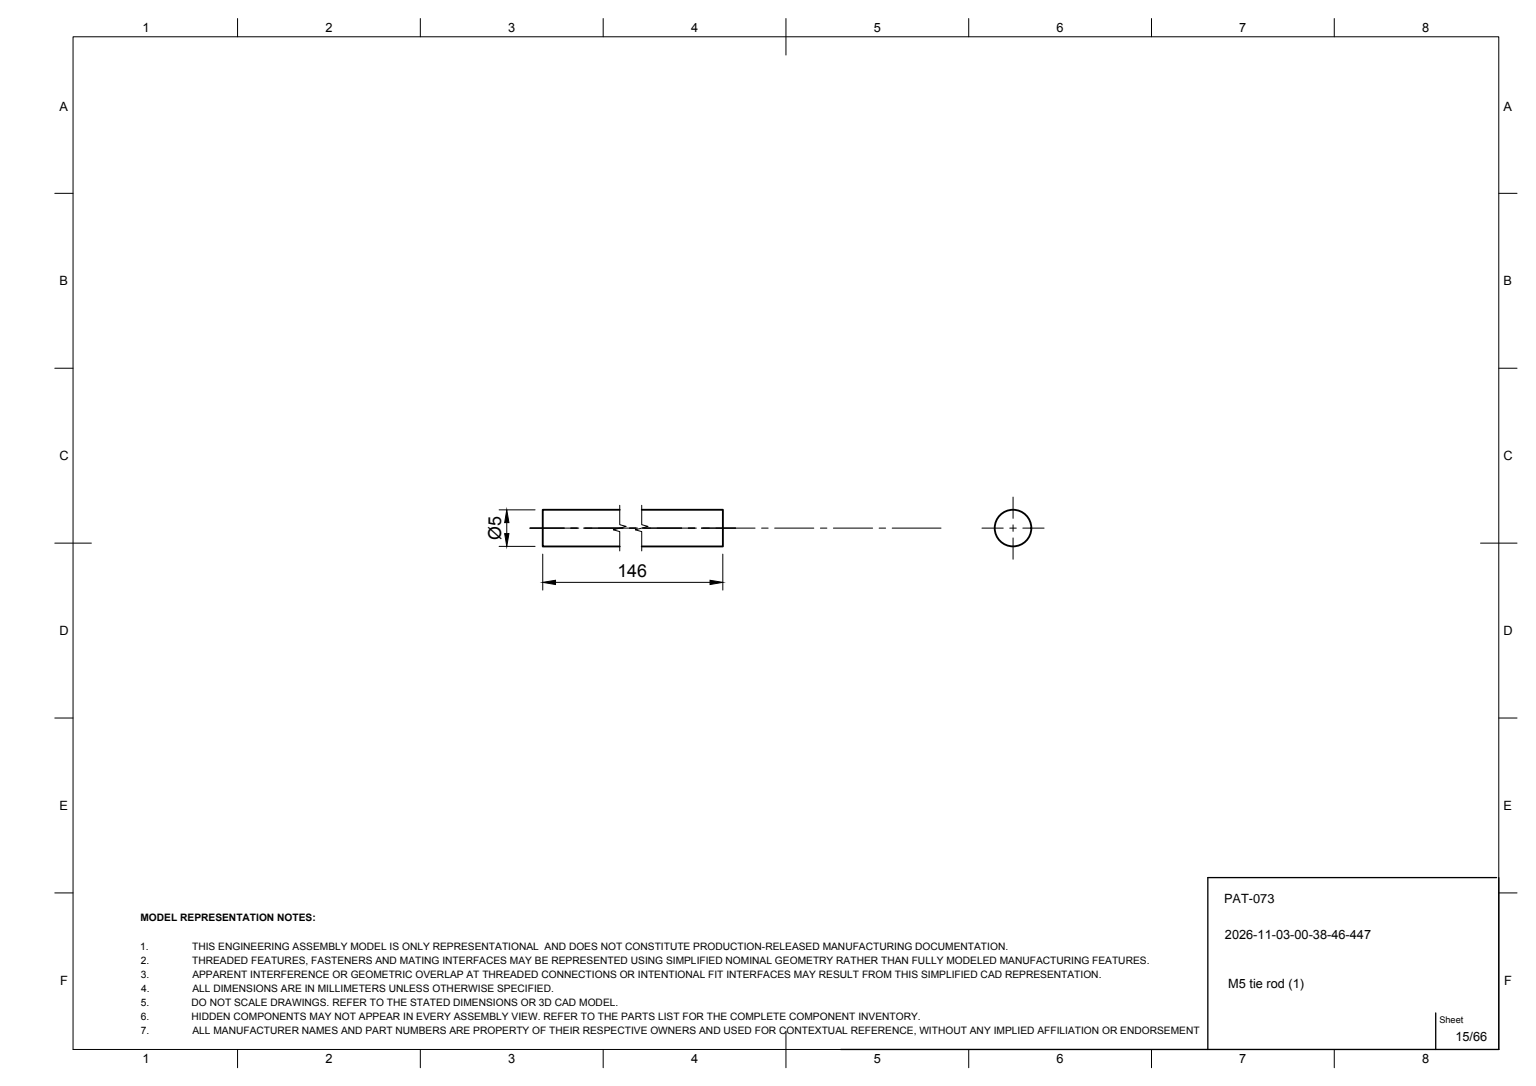
ISO-10303-21;
HEADER;
/* Generated by software containing ST-Developer
 * from STEP Tools, Inc. (www.steptools.com) 
 */

FILE_DESCRIPTION(
/* description */ ('Manual piston pump'),
/* implementation_level */ '2;1');

FILE_NAME(
/* name */ 'M5 tie rod (1).step',
/* time_stamp */ '2026-11-02T16:54:23-08:00',
/* author */ (''),
/* organization */ (''),
/* preprocessor_version */ 'ST-DEVELOPER v20.2',
/* originating_system */ 'Autodesk Translation Framework v15.17.0.0',
/* authorisation */ '');

FILE_SCHEMA (('AUTOMOTIVE_DESIGN { 1 0 10303 214 3 1 1 }'));
ENDSEC;

DATA;
#10=MECHANICAL_DESIGN_GEOMETRIC_PRESENTATION_REPRESENTATION('',(#698),#19043);
#572=SHAPE_REPRESENTATION_RELATIONSHIP('SRR','None',#19318,#635);
#635=ADVANCED_BREP_SHAPE_REPRESENTATION('',(#770),#18985);
#698=STYLED_ITEM('',(#19661),#770);
#770=MANIFOLD_SOLID_BREP('Body1',#9482);
#1139=CYLINDRICAL_SURFACE('',#10460,0.25);
#1396=FACE_OUTER_BOUND('',#2028,.T.);
#1397=FACE_OUTER_BOUND('',#2029,.T.);
#1398=FACE_OUTER_BOUND('',#2030,.T.);
#2028=EDGE_LOOP('',(#6717,#6718,#6719,#6720));
#2029=EDGE_LOOP('',(#6721));
#2030=EDGE_LOOP('',(#6722));
#2763=CIRCLE('',#10461,0.25);
#2764=CIRCLE('',#10462,0.25);
#3266=LINE('',#15144,#3870);
#3870=VECTOR('',#12052,0.25);
#4502=VERTEX_POINT('',#15141);
#4503=VERTEX_POINT('',#15143);
#5345=EDGE_CURVE('',#4502,#4502,#2763,.T.);
#5346=EDGE_CURVE('',#4502,#4503,#3266,.T.);
#5347=EDGE_CURVE('',#4503,#4503,#2764,.T.);
#6717=ORIENTED_EDGE('',*,*,#5345,.F.);
#6718=ORIENTED_EDGE('',*,*,#5346,.T.);
#6719=ORIENTED_EDGE('',*,*,#5347,.T.);
#6720=ORIENTED_EDGE('',*,*,#5346,.F.);
#6721=ORIENTED_EDGE('',*,*,#5345,.T.);
#6722=ORIENTED_EDGE('',*,*,#5347,.F.);
#8628=PLANE('',#10463);
#8629=PLANE('',#10464);
#9001=ADVANCED_FACE('',(#1396),#1139,.T.);
#9002=ADVANCED_FACE('',(#1397),#8628,.T.);
#9003=ADVANCED_FACE('',(#1398),#8629,.F.);
#9482=CLOSED_SHELL('',(#9001,#9002,#9003));
#10459=AXIS2_PLACEMENT_3D('',#15139,#12046,#12047);
#10460=AXIS2_PLACEMENT_3D('',#15140,#12048,#12049);
#10461=AXIS2_PLACEMENT_3D('',#15142,#12050,#12051);
#10462=AXIS2_PLACEMENT_3D('',#15145,#12053,#12054);
#10463=AXIS2_PLACEMENT_3D('',#15146,#12055,#12056);
#10464=AXIS2_PLACEMENT_3D('',#15147,#12057,#12058);
#12046=DIRECTION('axis',(0.,0.,1.));
#12047=DIRECTION('refdir',(1.,0.,0.));
#12048=DIRECTION('center_axis',(0.,1.,0.));
#12049=DIRECTION('ref_axis',(1.,0.,0.));
#12050=DIRECTION('center_axis',(0.,1.,0.));
#12051=DIRECTION('ref_axis',(1.,0.,0.));
#12052=DIRECTION('',(0.,-1.,0.));
#12053=DIRECTION('center_axis',(0.,1.,0.));
#12054=DIRECTION('ref_axis',(1.,0.,0.));
#12055=DIRECTION('center_axis',(0.,1.,0.));
#12056=DIRECTION('ref_axis',(1.,0.,0.));
#12057=DIRECTION('center_axis',(0.,1.,0.));
#12058=DIRECTION('ref_axis',(1.,0.,0.));
#15139=CARTESIAN_POINT('',(0.,0.,0.));
#15140=CARTESIAN_POINT('Origin',(-2.,-1.,6.5));
#15141=CARTESIAN_POINT('',(-2.25,13.6,6.5));
#15142=CARTESIAN_POINT('Origin',(-2.,13.6,6.5));
#15143=CARTESIAN_POINT('',(-2.25,-1.,6.5));
#15144=CARTESIAN_POINT('',(-2.25,-1.,6.5));
#15145=CARTESIAN_POINT('Origin',(-2.,-1.,6.5));
#15146=CARTESIAN_POINT('Origin',(-2.,13.6,6.5));
#15147=CARTESIAN_POINT('Origin',(-2.,-1.,6.5));
#18914=UNCERTAINTY_MEASURE_WITH_UNIT(LENGTH_MEASURE(0.001),#19044,
'DISTANCE_ACCURACY_VALUE',
'Maximum model space distance between geometric entities at asserted c
onnectivities');
#18972=UNCERTAINTY_MEASURE_WITH_UNIT(LENGTH_MEASURE(0.001),#19044,
'DISTANCE_ACCURACY_VALUE',
'Maximum model space distance between geometric entities at asserted c
onnectivities');
#18985=(
GEOMETRIC_REPRESENTATION_CONTEXT(3)
GLOBAL_UNCERTAINTY_ASSIGNED_CONTEXT((#18914))
GLOBAL_UNIT_ASSIGNED_CONTEXT((#19044,#19046,#19047))
REPRESENTATION_CONTEXT('','3D')
);
#19043=(
GEOMETRIC_REPRESENTATION_CONTEXT(3)
GLOBAL_UNCERTAINTY_ASSIGNED_CONTEXT((#18972))
GLOBAL_UNIT_ASSIGNED_CONTEXT((#19044,#19046,#19047))
REPRESENTATION_CONTEXT('','3D')
);
#19044=(
LENGTH_UNIT()
NAMED_UNIT(*)
SI_UNIT(.CENTI.,.METRE.)
);
#19046=(
NAMED_UNIT(*)
PLANE_ANGLE_UNIT()
SI_UNIT($,.RADIAN.)
);
#19047=(
NAMED_UNIT(*)
SI_UNIT($,.STERADIAN.)
SOLID_ANGLE_UNIT()
);
#19060=SHAPE_DEFINITION_REPRESENTATION(#19130,#19318);
#19130=PRODUCT_DEFINITION_SHAPE('',$,#19389);
#19318=SHAPE_REPRESENTATION('',(#10459),#18985);
#19376=PRODUCT_DEFINITION_CONTEXT('part definition',#19588,'design');
#19389=PRODUCT_DEFINITION('2026-11-03-00-38-46-447','M5 tie rod (1)',#19459,
#19376);
#19459=PRODUCT_DEFINITION_FORMATION('',$,#19602);
#19588=APPLICATION_CONTEXT(
'Core Data for Automotive Mechanical Design Process');
#19589=PRODUCT_CONTEXT('part definition',#19588,'mechanical');
#19602=PRODUCT('2026-11-03-00-38-46-447','M5 tie rod (1)','M5 tie rod',
(#19589));
#19661=PRESENTATION_STYLE_ASSIGNMENT((#19667));
#19667=SURFACE_STYLE_USAGE(.BOTH.,#19673);
#19673=SURFACE_SIDE_STYLE('',(#19679));
#19679=SURFACE_STYLE_FILL_AREA(#19685);
#19685=FILL_AREA_STYLE('CAD Library Painted - Engineering blue',(#19691));
#19691=FILL_AREA_STYLE_COLOUR('CAD Library Painted - Engineering blue',
#19697);
#19697=COLOUR_RGB('CAD Library Painted - Engineering blue',0.12156862745098,
0.356862745098039,0.6);
ENDSEC;
END-ISO-10303-21;
